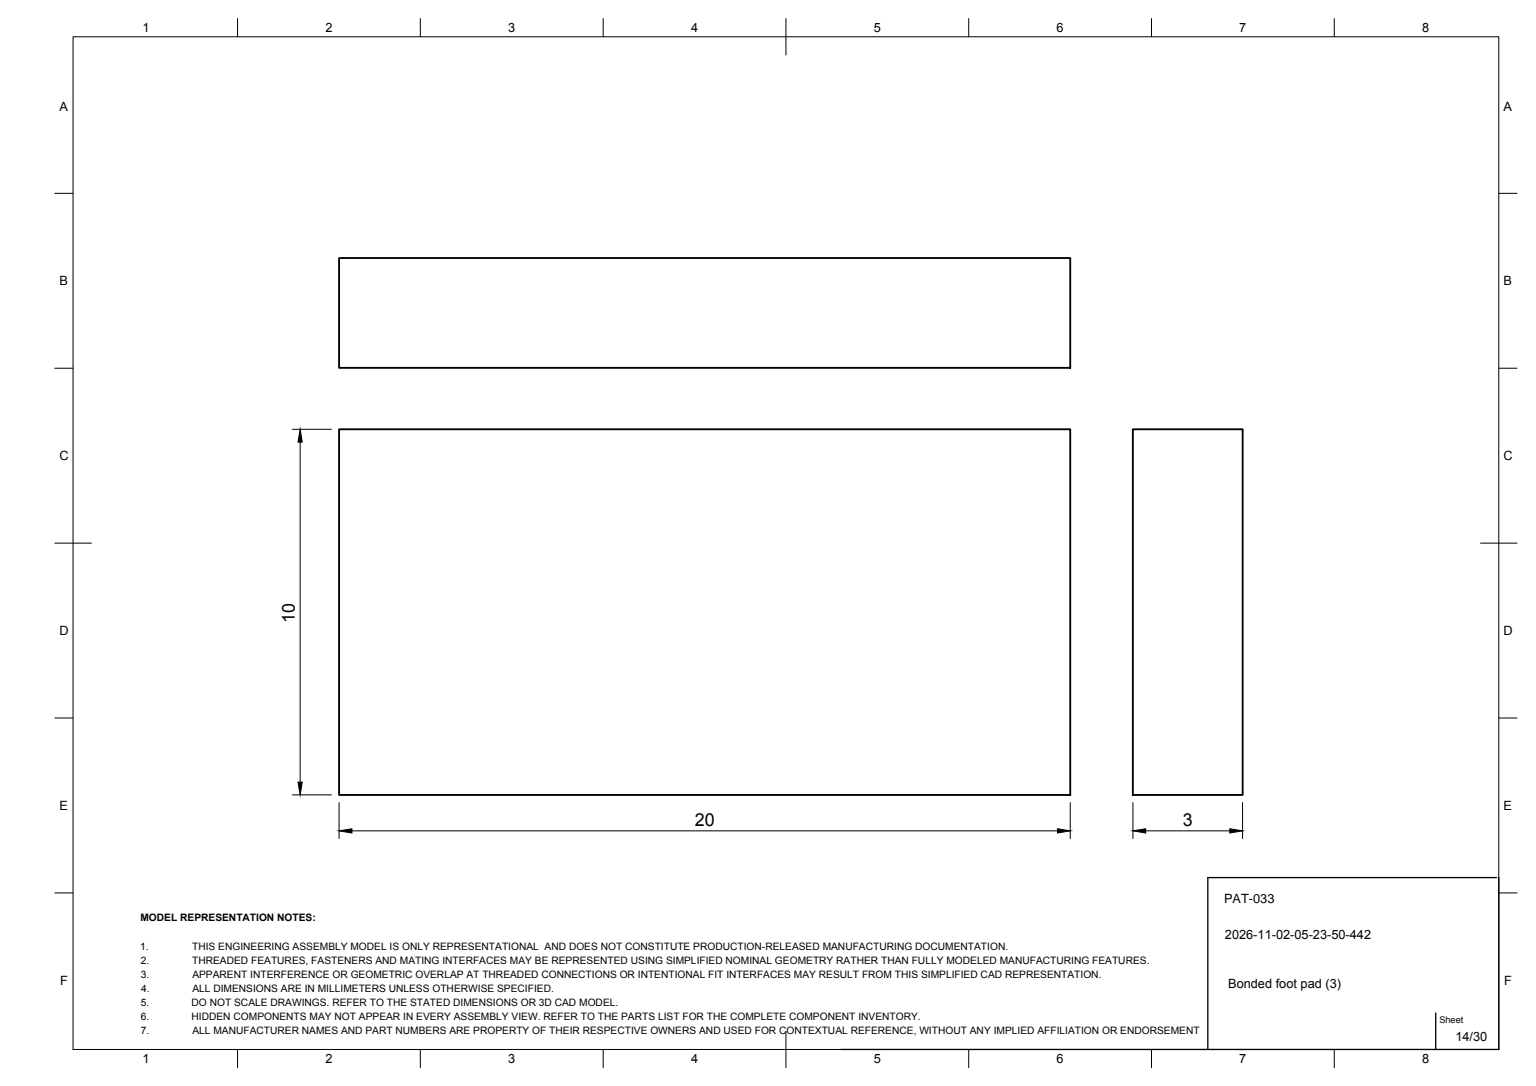
ISO-10303-21;
HEADER;
/* Generated by software containing ST-Developer
 * from STEP Tools, Inc. (www.steptools.com) 
 */

FILE_DESCRIPTION(
/* description */ ('Dual-rail gantry carriage'),
/* implementation_level */ '2;1');

FILE_NAME(
/* name */ 'Bonded foot pad (3).step',
/* time_stamp */ '2026-10-27T10:49:15-07:00',
/* author */ (''),
/* organization */ (''),
/* preprocessor_version */ 'ST-DEVELOPER v20.2',
/* originating_system */ 'Autodesk Translation Framework v15.17.0.0',
/* authorisation */ '');

FILE_SCHEMA (('AUTOMOTIVE_DESIGN { 1 0 10303 214 3 1 1 }'));
ENDSEC;

DATA;
#10=MECHANICAL_DESIGN_GEOMETRIC_PRESENTATION_REPRESENTATION('',(#594),#12804);
#532=SHAPE_REPRESENTATION_RELATIONSHIP('SRR','None',#13010,#563);
#563=ADVANCED_BREP_SHAPE_REPRESENTATION('',(#625),#12780);
#594=STYLED_ITEM('',(#13240),#625);
#625=MANIFOLD_SOLID_BREP('Body1',#7372);
#818=PLANE('',#7867);
#819=PLANE('',#7868);
#820=PLANE('',#7869);
#821=PLANE('',#7870);
#822=PLANE('',#7871);
#823=PLANE('',#7872);
#1122=FACE_OUTER_BOUND('',#1551,.T.);
#1123=FACE_OUTER_BOUND('',#1552,.T.);
#1124=FACE_OUTER_BOUND('',#1553,.T.);
#1125=FACE_OUTER_BOUND('',#1554,.T.);
#1126=FACE_OUTER_BOUND('',#1555,.T.);
#1127=FACE_OUTER_BOUND('',#1556,.T.);
#1551=EDGE_LOOP('',(#5403,#5404,#5405,#5406));
#1552=EDGE_LOOP('',(#5407,#5408,#5409,#5410));
#1553=EDGE_LOOP('',(#5411,#5412,#5413,#5414));
#1554=EDGE_LOOP('',(#5415,#5416,#5417,#5418));
#1555=EDGE_LOOP('',(#5419,#5420,#5421,#5422));
#1556=EDGE_LOOP('',(#5423,#5424,#5425,#5426));
#2076=LINE('',#11057,#2785);
#2077=LINE('',#11059,#2786);
#2078=LINE('',#11061,#2787);
#2079=LINE('',#11062,#2788);
#2080=LINE('',#11065,#2789);
#2081=LINE('',#11067,#2790);
#2082=LINE('',#11068,#2791);
#2083=LINE('',#11071,#2792);
#2084=LINE('',#11073,#2793);
#2085=LINE('',#11074,#2794);
#2086=LINE('',#11076,#2795);
#2087=LINE('',#11077,#2796);
#2785=VECTOR('',#8869,1.);
#2786=VECTOR('',#8870,1.);
#2787=VECTOR('',#8871,1.);
#2788=VECTOR('',#8872,1.);
#2789=VECTOR('',#8875,1.);
#2790=VECTOR('',#8876,1.);
#2791=VECTOR('',#8877,1.);
#2792=VECTOR('',#8880,1.);
#2793=VECTOR('',#8881,1.);
#2794=VECTOR('',#8882,1.);
#2795=VECTOR('',#8885,1.);
#2796=VECTOR('',#8886,1.);
#3678=VERTEX_POINT('',#11055);
#3679=VERTEX_POINT('',#11056);
#3680=VERTEX_POINT('',#11058);
#3681=VERTEX_POINT('',#11060);
#3682=VERTEX_POINT('',#11064);
#3683=VERTEX_POINT('',#11066);
#3684=VERTEX_POINT('',#11070);
#3685=VERTEX_POINT('',#11072);
#4324=EDGE_CURVE('',#3678,#3679,#2076,.T.);
#4325=EDGE_CURVE('',#3679,#3680,#2077,.T.);
#4326=EDGE_CURVE('',#3681,#3680,#2078,.T.);
#4327=EDGE_CURVE('',#3678,#3681,#2079,.T.);
#4328=EDGE_CURVE('',#3682,#3678,#2080,.T.);
#4329=EDGE_CURVE('',#3683,#3681,#2081,.T.);
#4330=EDGE_CURVE('',#3682,#3683,#2082,.T.);
#4331=EDGE_CURVE('',#3684,#3682,#2083,.T.);
#4332=EDGE_CURVE('',#3685,#3683,#2084,.T.);
#4333=EDGE_CURVE('',#3684,#3685,#2085,.T.);
#4334=EDGE_CURVE('',#3679,#3684,#2086,.T.);
#4335=EDGE_CURVE('',#3680,#3685,#2087,.T.);
#5403=ORIENTED_EDGE('',*,*,#4324,.T.);
#5404=ORIENTED_EDGE('',*,*,#4325,.T.);
#5405=ORIENTED_EDGE('',*,*,#4326,.F.);
#5406=ORIENTED_EDGE('',*,*,#4327,.F.);
#5407=ORIENTED_EDGE('',*,*,#4328,.T.);
#5408=ORIENTED_EDGE('',*,*,#4327,.T.);
#5409=ORIENTED_EDGE('',*,*,#4329,.F.);
#5410=ORIENTED_EDGE('',*,*,#4330,.F.);
#5411=ORIENTED_EDGE('',*,*,#4331,.T.);
#5412=ORIENTED_EDGE('',*,*,#4330,.T.);
#5413=ORIENTED_EDGE('',*,*,#4332,.F.);
#5414=ORIENTED_EDGE('',*,*,#4333,.F.);
#5415=ORIENTED_EDGE('',*,*,#4334,.T.);
#5416=ORIENTED_EDGE('',*,*,#4333,.T.);
#5417=ORIENTED_EDGE('',*,*,#4335,.F.);
#5418=ORIENTED_EDGE('',*,*,#4325,.F.);
#5419=ORIENTED_EDGE('',*,*,#4335,.T.);
#5420=ORIENTED_EDGE('',*,*,#4332,.T.);
#5421=ORIENTED_EDGE('',*,*,#4329,.T.);
#5422=ORIENTED_EDGE('',*,*,#4326,.T.);
#5423=ORIENTED_EDGE('',*,*,#4334,.F.);
#5424=ORIENTED_EDGE('',*,*,#4324,.F.);
#5425=ORIENTED_EDGE('',*,*,#4328,.F.);
#5426=ORIENTED_EDGE('',*,*,#4331,.F.);
#7048=ADVANCED_FACE('',(#1122),#818,.T.);
#7049=ADVANCED_FACE('',(#1123),#819,.T.);
#7050=ADVANCED_FACE('',(#1124),#820,.T.);
#7051=ADVANCED_FACE('',(#1125),#821,.T.);
#7052=ADVANCED_FACE('',(#1126),#822,.T.);
#7053=ADVANCED_FACE('',(#1127),#823,.F.);
#7372=CLOSED_SHELL('',(#7048,#7049,#7050,#7051,#7052,#7053));
#7866=AXIS2_PLACEMENT_3D('',#11053,#8865,#8866);
#7867=AXIS2_PLACEMENT_3D('',#11054,#8867,#8868);
#7868=AXIS2_PLACEMENT_3D('',#11063,#8873,#8874);
#7869=AXIS2_PLACEMENT_3D('',#11069,#8878,#8879);
#7870=AXIS2_PLACEMENT_3D('',#11075,#8883,#8884);
#7871=AXIS2_PLACEMENT_3D('',#11078,#8887,#8888);
#7872=AXIS2_PLACEMENT_3D('',#11079,#8889,#8890);
#8865=DIRECTION('axis',(0.,0.,1.));
#8866=DIRECTION('refdir',(1.,0.,0.));
#8867=DIRECTION('center_axis',(0.,1.,0.));
#8868=DIRECTION('ref_axis',(-1.,0.,0.));
#8869=DIRECTION('',(-1.,0.,0.));
#8870=DIRECTION('',(0.,0.,1.));
#8871=DIRECTION('',(-1.,0.,0.));
#8872=DIRECTION('',(0.,0.,1.));
#8873=DIRECTION('center_axis',(1.,0.,0.));
#8874=DIRECTION('ref_axis',(0.,1.,0.));
#8875=DIRECTION('',(0.,1.,0.));
#8876=DIRECTION('',(0.,1.,0.));
#8877=DIRECTION('',(0.,0.,1.));
#8878=DIRECTION('center_axis',(0.,-1.,0.));
#8879=DIRECTION('ref_axis',(1.,0.,0.));
#8880=DIRECTION('',(1.,0.,0.));
#8881=DIRECTION('',(1.,0.,0.));
#8882=DIRECTION('',(0.,0.,1.));
#8883=DIRECTION('center_axis',(-1.,0.,0.));
#8884=DIRECTION('ref_axis',(0.,-1.,0.));
#8885=DIRECTION('',(0.,-1.,0.));
#8886=DIRECTION('',(0.,-1.,0.));
#8887=DIRECTION('center_axis',(0.,0.,1.));
#8888=DIRECTION('ref_axis',(1.,0.,0.));
#8889=DIRECTION('center_axis',(0.,0.,1.));
#8890=DIRECTION('ref_axis',(1.,0.,0.));
#11053=CARTESIAN_POINT('',(0.,0.,0.));
#11054=CARTESIAN_POINT('Origin',(40.,12.5,-1.1));
#11055=CARTESIAN_POINT('',(40.,12.5,-1.1));
#11056=CARTESIAN_POINT('',(38.,12.5,-1.1));
#11057=CARTESIAN_POINT('',(40.,12.5,-1.1));
#11058=CARTESIAN_POINT('',(38.,12.5,-0.8));
#11059=CARTESIAN_POINT('',(38.,12.5,-1.1));
#11060=CARTESIAN_POINT('',(40.,12.5,-0.8));
#11061=CARTESIAN_POINT('',(40.,12.5,-0.8));
#11062=CARTESIAN_POINT('',(40.,12.5,-1.1));
#11063=CARTESIAN_POINT('Origin',(40.,11.5,-1.1));
#11064=CARTESIAN_POINT('',(40.,11.5,-1.1));
#11065=CARTESIAN_POINT('',(40.,11.5,-1.1));
#11066=CARTESIAN_POINT('',(40.,11.5,-0.8));
#11067=CARTESIAN_POINT('',(40.,11.5,-0.8));
#11068=CARTESIAN_POINT('',(40.,11.5,-1.1));
#11069=CARTESIAN_POINT('Origin',(38.,11.5,-1.1));
#11070=CARTESIAN_POINT('',(38.,11.5,-1.1));
#11071=CARTESIAN_POINT('',(38.,11.5,-1.1));
#11072=CARTESIAN_POINT('',(38.,11.5,-0.8));
#11073=CARTESIAN_POINT('',(38.,11.5,-0.8));
#11074=CARTESIAN_POINT('',(38.,11.5,-1.1));
#11075=CARTESIAN_POINT('Origin',(38.,12.5,-1.1));
#11076=CARTESIAN_POINT('',(38.,12.5,-1.1));
#11077=CARTESIAN_POINT('',(38.,12.5,-0.8));
#11078=CARTESIAN_POINT('Origin',(39.,12.,-0.8));
#11079=CARTESIAN_POINT('Origin',(39.,12.,-1.1));
#12744=UNCERTAINTY_MEASURE_WITH_UNIT(LENGTH_MEASURE(0.001),#12805,
'DISTANCE_ACCURACY_VALUE',
'Maximum model space distance between geometric entities at asserted c
onnectivities');
#12768=UNCERTAINTY_MEASURE_WITH_UNIT(LENGTH_MEASURE(0.001),#12805,
'DISTANCE_ACCURACY_VALUE',
'Maximum model space distance between geometric entities at asserted c
onnectivities');
#12780=(
GEOMETRIC_REPRESENTATION_CONTEXT(3)
GLOBAL_UNCERTAINTY_ASSIGNED_CONTEXT((#12744))
GLOBAL_UNIT_ASSIGNED_CONTEXT((#12805,#12807,#12808))
REPRESENTATION_CONTEXT('','3D')
);
#12804=(
GEOMETRIC_REPRESENTATION_CONTEXT(3)
GLOBAL_UNCERTAINTY_ASSIGNED_CONTEXT((#12768))
GLOBAL_UNIT_ASSIGNED_CONTEXT((#12805,#12807,#12808))
REPRESENTATION_CONTEXT('','3D')
);
#12805=(
LENGTH_UNIT()
NAMED_UNIT(*)
SI_UNIT(.CENTI.,.METRE.)
);
#12807=(
NAMED_UNIT(*)
PLANE_ANGLE_UNIT()
SI_UNIT($,.RADIAN.)
);
#12808=(
NAMED_UNIT(*)
SI_UNIT($,.STERADIAN.)
SOLID_ANGLE_UNIT()
);
#12820=SHAPE_DEFINITION_REPRESENTATION(#12855,#13010);
#12855=PRODUCT_DEFINITION_SHAPE('',$,#13046);
#13010=SHAPE_REPRESENTATION('',(#7866),#12780);
#13034=PRODUCT_DEFINITION_CONTEXT('part definition',#13141,'design');
#13046=PRODUCT_DEFINITION('Bonded foot pad (3)','Bonded foot pad (3)',#13081,
#13034);
#13081=PRODUCT_DEFINITION_FORMATION('',$,#13154);
#13141=APPLICATION_CONTEXT(
'Core Data for Automotive Mechanical Design Process');
#13142=PRODUCT_CONTEXT('part definition',#13141,'mechanical');
#13154=PRODUCT('Bonded foot pad (3)','Bonded foot pad (3)',
'Bonded foot pad (3)',(#13142));
#13234=COLOUR_RGB('Sky Blue',0.24,0.69,0.87);
#13235=FILL_AREA_STYLE_COLOUR('',#13234);
#13236=FILL_AREA_STYLE('',(#13235));
#13237=SURFACE_STYLE_FILL_AREA(#13236);
#13238=SURFACE_SIDE_STYLE('',(#13237));
#13239=SURFACE_STYLE_USAGE(.BOTH.,#13238);
#13240=PRESENTATION_STYLE_ASSIGNMENT((#13239));
ENDSEC;
END-ISO-10303-21;
